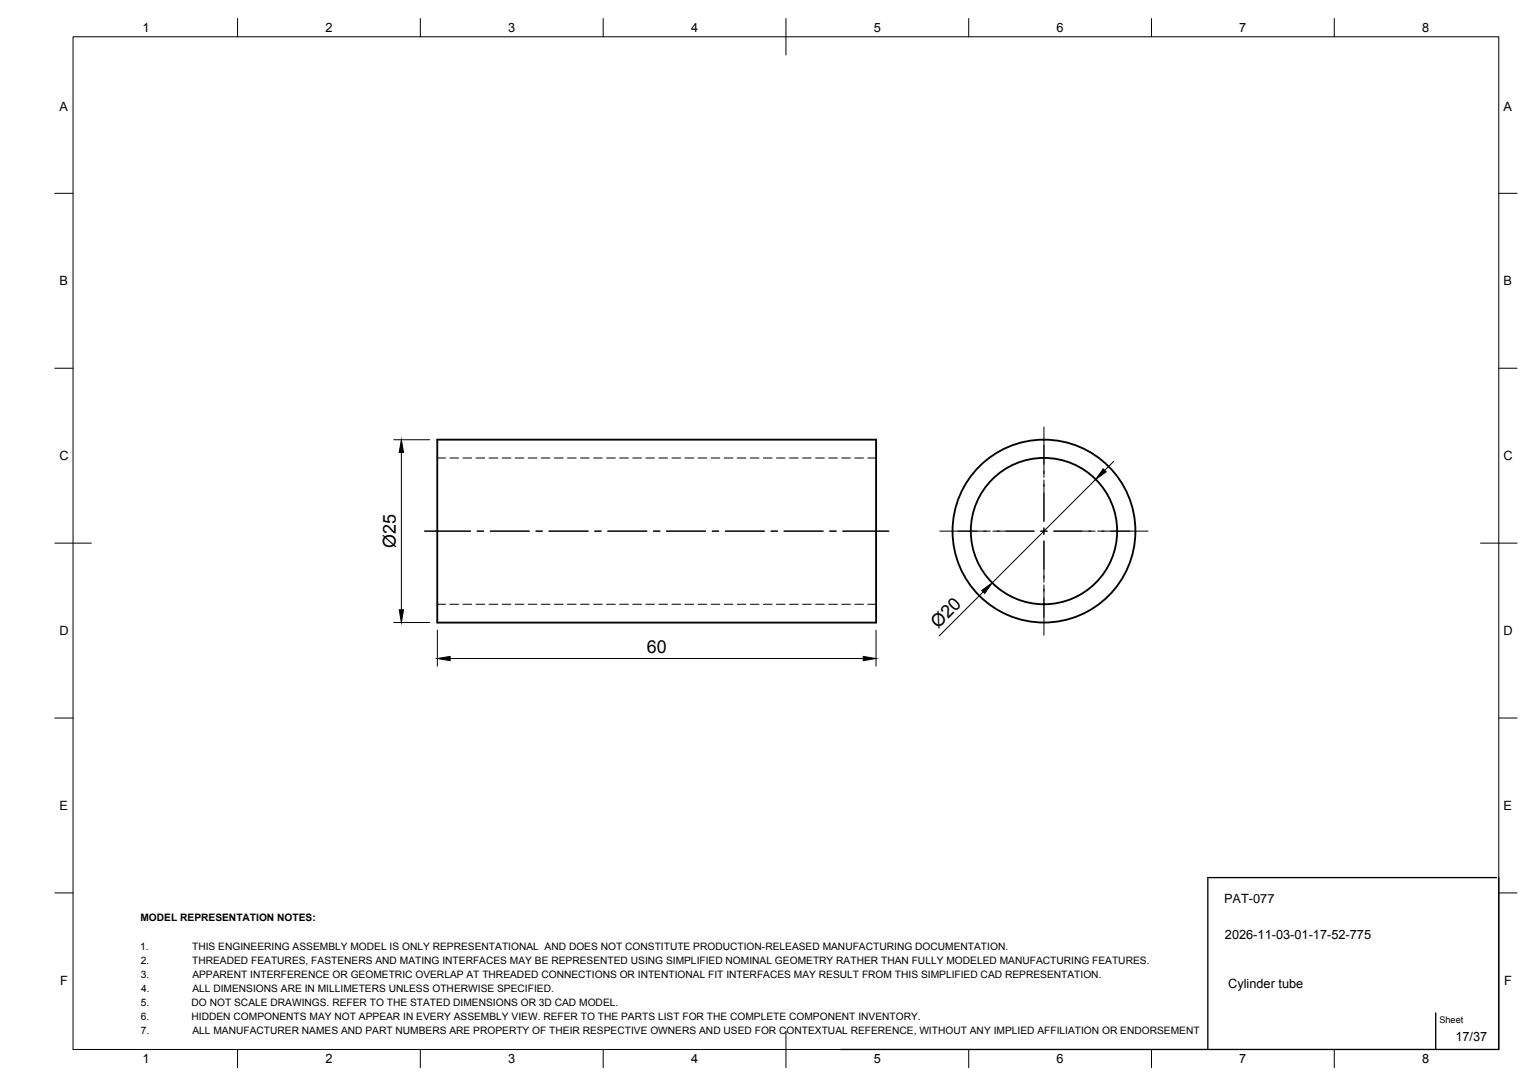
ISO-10303-21;
HEADER;
/* Generated by software containing ST-Developer
 * from STEP Tools, Inc. (www.steptools.com) 
 */

FILE_DESCRIPTION(
/* description */ ('Pallet stop with pneumatic fitting'),
/* implementation_level */ '2;1');

FILE_NAME(
/* name */ 'Cylinder tube.step',
/* time_stamp */ '2026-10-27T10:51:41-07:00',
/* author */ (''),
/* organization */ (''),
/* preprocessor_version */ 'ST-DEVELOPER v20.2',
/* originating_system */ 'Autodesk Translation Framework v15.17.0.0',
/* authorisation */ '');

FILE_SCHEMA (('AUTOMOTIVE_DESIGN { 1 0 10303 214 3 1 1 }'));
ENDSEC;

DATA;
#10=MECHANICAL_DESIGN_GEOMETRIC_PRESENTATION_REPRESENTATION('',(#369),#10265);
#305=SHAPE_REPRESENTATION_RELATIONSHIP('SRR','None',#10418,#337);
#337=ADVANCED_BREP_SHAPE_REPRESENTATION('',(#401),#10242);
#369=STYLED_ITEM('',(#10648),#401);
#401=MANIFOLD_SOLID_BREP('Body1',#5057);
#500=FACE_BOUND('',#1272,.T.);
#501=FACE_BOUND('',#1274,.T.);
#620=PLANE('',#5716);
#621=PLANE('',#5717);
#874=FACE_OUTER_BOUND('',#1269,.T.);
#875=FACE_OUTER_BOUND('',#1270,.T.);
#876=FACE_OUTER_BOUND('',#1271,.T.);
#877=FACE_OUTER_BOUND('',#1273,.T.);
#1269=EDGE_LOOP('',(#3952,#3953,#3954,#3955));
#1270=EDGE_LOOP('',(#3956,#3957,#3958,#3959));
#1271=EDGE_LOOP('',(#3960));
#1272=EDGE_LOOP('',(#3961));
#1273=EDGE_LOOP('',(#3962));
#1274=EDGE_LOOP('',(#3963));
#1628=LINE('',#9298,#1963);
#1629=LINE('',#9304,#1964);
#1963=VECTOR('',#6787,1.);
#1964=VECTOR('',#6794,1.25);
#2286=CIRCLE('',#5711,1.);
#2287=CIRCLE('',#5712,1.);
#2288=CIRCLE('',#5714,1.25);
#2289=CIRCLE('',#5715,1.25);
#2586=VERTEX_POINT('',#9295);
#2587=VERTEX_POINT('',#9297);
#2588=VERTEX_POINT('',#9301);
#2589=VERTEX_POINT('',#9303);
#3075=EDGE_CURVE('',#2586,#2586,#2286,.T.);
#3076=EDGE_CURVE('',#2586,#2587,#1628,.T.);
#3077=EDGE_CURVE('',#2587,#2587,#2287,.T.);
#3078=EDGE_CURVE('',#2588,#2588,#2288,.T.);
#3079=EDGE_CURVE('',#2588,#2589,#1629,.T.);
#3080=EDGE_CURVE('',#2589,#2589,#2289,.T.);
#3952=ORIENTED_EDGE('',*,*,#3075,.F.);
#3953=ORIENTED_EDGE('',*,*,#3076,.T.);
#3954=ORIENTED_EDGE('',*,*,#3077,.T.);
#3955=ORIENTED_EDGE('',*,*,#3076,.F.);
#3956=ORIENTED_EDGE('',*,*,#3078,.F.);
#3957=ORIENTED_EDGE('',*,*,#3079,.T.);
#3958=ORIENTED_EDGE('',*,*,#3080,.T.);
#3959=ORIENTED_EDGE('',*,*,#3079,.F.);
#3960=ORIENTED_EDGE('',*,*,#3078,.T.);
#3961=ORIENTED_EDGE('',*,*,#3075,.T.);
#3962=ORIENTED_EDGE('',*,*,#3080,.F.);
#3963=ORIENTED_EDGE('',*,*,#3077,.F.);
#4684=CYLINDRICAL_SURFACE('',#5710,1.);
#4685=CYLINDRICAL_SURFACE('',#5713,1.25);
#4869=ADVANCED_FACE('',(#874),#4684,.F.);
#4870=ADVANCED_FACE('',(#875),#4685,.T.);
#4871=ADVANCED_FACE('',(#876,#500),#620,.T.);
#4872=ADVANCED_FACE('',(#877,#501),#621,.F.);
#5057=CLOSED_SHELL('',(#4869,#4870,#4871,#4872));
#5709=AXIS2_PLACEMENT_3D('',#9293,#6781,#6782);
#5710=AXIS2_PLACEMENT_3D('',#9294,#6783,#6784);
#5711=AXIS2_PLACEMENT_3D('',#9296,#6785,#6786);
#5712=AXIS2_PLACEMENT_3D('',#9299,#6788,#6789);
#5713=AXIS2_PLACEMENT_3D('',#9300,#6790,#6791);
#5714=AXIS2_PLACEMENT_3D('',#9302,#6792,#6793);
#5715=AXIS2_PLACEMENT_3D('',#9305,#6795,#6796);
#5716=AXIS2_PLACEMENT_3D('',#9306,#6797,#6798);
#5717=AXIS2_PLACEMENT_3D('',#9307,#6799,#6800);
#6781=DIRECTION('axis',(0.,0.,1.));
#6782=DIRECTION('refdir',(1.,0.,0.));
#6783=DIRECTION('center_axis',(0.,0.,1.));
#6784=DIRECTION('ref_axis',(1.,0.,0.));
#6785=DIRECTION('center_axis',(0.,0.,-1.));
#6786=DIRECTION('ref_axis',(1.,0.,0.));
#6787=DIRECTION('',(0.,0.,-1.));
#6788=DIRECTION('center_axis',(0.,0.,-1.));
#6789=DIRECTION('ref_axis',(1.,0.,0.));
#6790=DIRECTION('center_axis',(0.,0.,1.));
#6791=DIRECTION('ref_axis',(1.,0.,0.));
#6792=DIRECTION('center_axis',(0.,0.,1.));
#6793=DIRECTION('ref_axis',(1.,0.,0.));
#6794=DIRECTION('',(0.,0.,-1.));
#6795=DIRECTION('center_axis',(0.,0.,1.));
#6796=DIRECTION('ref_axis',(1.,0.,0.));
#6797=DIRECTION('center_axis',(0.,0.,1.));
#6798=DIRECTION('ref_axis',(1.,0.,0.));
#6799=DIRECTION('center_axis',(0.,0.,1.));
#6800=DIRECTION('ref_axis',(1.,0.,0.));
#9293=CARTESIAN_POINT('',(0.,0.,0.));
#9294=CARTESIAN_POINT('Origin',(4.,4.,2.));
#9295=CARTESIAN_POINT('',(3.,4.,8.));
#9296=CARTESIAN_POINT('Origin',(4.,4.,8.));
#9297=CARTESIAN_POINT('',(3.,4.,2.));
#9298=CARTESIAN_POINT('',(3.,4.,2.));
#9299=CARTESIAN_POINT('Origin',(4.,4.,2.));
#9300=CARTESIAN_POINT('Origin',(4.,4.,2.));
#9301=CARTESIAN_POINT('',(2.75,4.,8.));
#9302=CARTESIAN_POINT('Origin',(4.,4.,8.));
#9303=CARTESIAN_POINT('',(2.75,4.,2.));
#9304=CARTESIAN_POINT('',(2.75,4.,2.));
#9305=CARTESIAN_POINT('Origin',(4.,4.,2.));
#9306=CARTESIAN_POINT('Origin',(4.,4.,8.));
#9307=CARTESIAN_POINT('Origin',(4.,4.,2.));
#10204=UNCERTAINTY_MEASURE_WITH_UNIT(LENGTH_MEASURE(0.001),#10266,
'DISTANCE_ACCURACY_VALUE',
'Maximum model space distance between geometric entities at asserted c
onnectivities');
#10227=UNCERTAINTY_MEASURE_WITH_UNIT(LENGTH_MEASURE(0.001),#10266,
'DISTANCE_ACCURACY_VALUE',
'Maximum model space distance between geometric entities at asserted c
onnectivities');
#10242=(
GEOMETRIC_REPRESENTATION_CONTEXT(3)
GLOBAL_UNCERTAINTY_ASSIGNED_CONTEXT((#10204))
GLOBAL_UNIT_ASSIGNED_CONTEXT((#10266,#10268,#10269))
REPRESENTATION_CONTEXT('','3D')
);
#10265=(
GEOMETRIC_REPRESENTATION_CONTEXT(3)
GLOBAL_UNCERTAINTY_ASSIGNED_CONTEXT((#10227))
GLOBAL_UNIT_ASSIGNED_CONTEXT((#10266,#10268,#10269))
REPRESENTATION_CONTEXT('','3D')
);
#10266=(
LENGTH_UNIT()
NAMED_UNIT(*)
SI_UNIT(.CENTI.,.METRE.)
);
#10268=(
NAMED_UNIT(*)
PLANE_ANGLE_UNIT()
SI_UNIT($,.RADIAN.)
);
#10269=(
NAMED_UNIT(*)
SI_UNIT($,.STERADIAN.)
SOLID_ANGLE_UNIT()
);
#10284=SHAPE_DEFINITION_REPRESENTATION(#10321,#10418);
#10321=PRODUCT_DEFINITION_SHAPE('',$,#10456);
#10418=SHAPE_REPRESENTATION('',(#5709),#10242);
#10441=PRODUCT_DEFINITION_CONTEXT('part definition',#10554,'design');
#10456=PRODUCT_DEFINITION('Cylinder tube','Cylinder tube',#10493,#10441);
#10493=PRODUCT_DEFINITION_FORMATION('',$,#10570);
#10554=APPLICATION_CONTEXT(
'Core Data for Automotive Mechanical Design Process');
#10555=PRODUCT_CONTEXT('part definition',#10554,'mechanical');
#10570=PRODUCT('Cylinder tube','Cylinder tube','Cylinder tube',(#10555));
#10642=COLOUR_RGB('Sky Blue',0.24,0.69,0.87);
#10643=FILL_AREA_STYLE_COLOUR('',#10642);
#10644=FILL_AREA_STYLE('',(#10643));
#10645=SURFACE_STYLE_FILL_AREA(#10644);
#10646=SURFACE_SIDE_STYLE('',(#10645));
#10647=SURFACE_STYLE_USAGE(.BOTH.,#10646);
#10648=PRESENTATION_STYLE_ASSIGNMENT((#10647));
ENDSEC;
END-ISO-10303-21;
